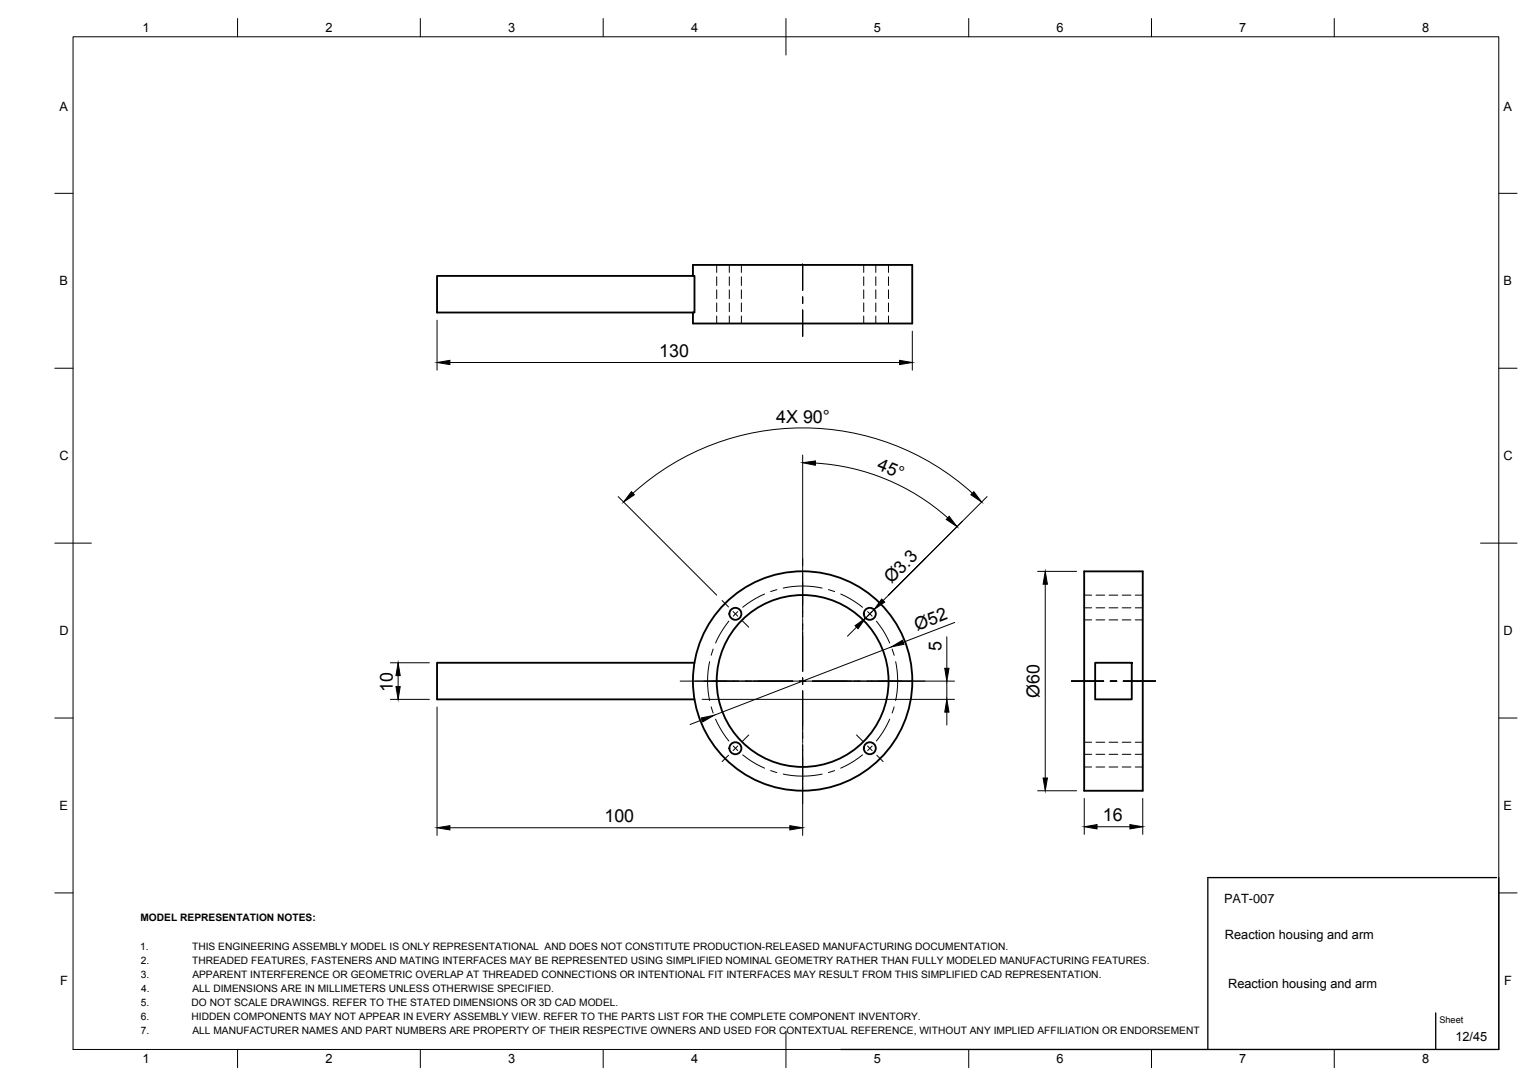
ISO-10303-21;
HEADER;
/* Generated by software containing ST-Developer
 * from STEP Tools, Inc. (www.steptools.com) 
 */

FILE_DESCRIPTION(
/* description */ ('Bearing friction torque test rig'),
/* implementation_level */ '2;1');

FILE_NAME(
/* name */ 'Reaction housing and arm.step',
/* time_stamp */ '2026-10-28T03:24:04-07:00',
/* author */ (''),
/* organization */ (''),
/* preprocessor_version */ 'ST-DEVELOPER v20.2',
/* originating_system */ 'Autodesk Translation Framework v15.17.0.0',
/* authorisation */ '');

FILE_SCHEMA (('AUTOMOTIVE_DESIGN { 1 0 10303 214 3 1 1 }'));
ENDSEC;

DATA;
#10=MECHANICAL_DESIGN_GEOMETRIC_PRESENTATION_REPRESENTATION('',(#546),#14822);
#468=SHAPE_REPRESENTATION_RELATIONSHIP('SRR','None',#15007,#507);
#507=ADVANCED_BREP_SHAPE_REPRESENTATION('',(#600),#14787);
#546=STYLED_ITEM('',(#15263),#600);
#600=MANIFOLD_SOLID_BREP('Body1',#7662);
#744=FACE_BOUND('',#1755,.T.);
#745=FACE_BOUND('',#1757,.T.);
#746=FACE_BOUND('',#1758,.T.);
#747=FACE_BOUND('',#1759,.T.);
#748=FACE_BOUND('',#1760,.T.);
#749=FACE_BOUND('',#1761,.T.);
#750=FACE_BOUND('',#1763,.T.);
#751=FACE_BOUND('',#1764,.T.);
#752=FACE_BOUND('',#1765,.T.);
#753=FACE_BOUND('',#1766,.T.);
#754=FACE_BOUND('',#1767,.T.);
#914=PLANE('',#8392);
#915=PLANE('',#8393);
#916=PLANE('',#8395);
#917=PLANE('',#8397);
#918=PLANE('',#8398);
#919=PLANE('',#8405);
#920=PLANE('',#8406);
#1199=FACE_OUTER_BOUND('',#1744,.T.);
#1200=FACE_OUTER_BOUND('',#1745,.T.);
#1201=FACE_OUTER_BOUND('',#1746,.T.);
#1202=FACE_OUTER_BOUND('',#1747,.T.);
#1203=FACE_OUTER_BOUND('',#1748,.T.);
#1204=FACE_OUTER_BOUND('',#1749,.T.);
#1205=FACE_OUTER_BOUND('',#1750,.T.);
#1206=FACE_OUTER_BOUND('',#1751,.T.);
#1207=FACE_OUTER_BOUND('',#1752,.T.);
#1208=FACE_OUTER_BOUND('',#1753,.T.);
#1209=FACE_OUTER_BOUND('',#1754,.T.);
#1210=FACE_OUTER_BOUND('',#1756,.T.);
#1211=FACE_OUTER_BOUND('',#1762,.T.);
#1744=EDGE_LOOP('',(#5616,#5617,#5618,#5619));
#1745=EDGE_LOOP('',(#5620,#5621,#5622,#5623));
#1746=EDGE_LOOP('',(#5624,#5625,#5626,#5627));
#1747=EDGE_LOOP('',(#5628,#5629,#5630,#5631));
#1748=EDGE_LOOP('',(#5632,#5633,#5634,#5635));
#1749=EDGE_LOOP('',(#5636,#5637,#5638,#5639));
#1750=EDGE_LOOP('',(#5640,#5641,#5642,#5643));
#1751=EDGE_LOOP('',(#5644,#5645,#5646,#5647));
#1752=EDGE_LOOP('',(#5648,#5649,#5650,#5651));
#1753=EDGE_LOOP('',(#5652,#5653,#5654,#5655));
#1754=EDGE_LOOP('',(#5656,#5657,#5658,#5659));
#1755=EDGE_LOOP('',(#5660,#5661,#5662,#5663));
#1756=EDGE_LOOP('',(#5664));
#1757=EDGE_LOOP('',(#5665));
#1758=EDGE_LOOP('',(#5666));
#1759=EDGE_LOOP('',(#5667));
#1760=EDGE_LOOP('',(#5668));
#1761=EDGE_LOOP('',(#5669));
#1762=EDGE_LOOP('',(#5670));
#1763=EDGE_LOOP('',(#5671));
#1764=EDGE_LOOP('',(#5672));
#1765=EDGE_LOOP('',(#5673));
#1766=EDGE_LOOP('',(#5674));
#1767=EDGE_LOOP('',(#5675));
#2325=LINE('',#12162,#2769);
#2326=LINE('',#12168,#2770);
#2327=LINE('',#12174,#2771);
#2328=LINE('',#12180,#2772);
#2329=LINE('',#12185,#2773);
#2330=LINE('',#12187,#2774);
#2331=LINE('',#12189,#2775);
#2332=LINE('',#12190,#2776);
#2333=LINE('',#12195,#2777);
#2334=LINE('',#12196,#2778);
#2335=LINE('',#12201,#2779);
#2336=LINE('',#12202,#2780);
#2337=LINE('',#12204,#2781);
#2338=LINE('',#12205,#2782);
#2339=LINE('',#12211,#2783);
#2340=LINE('',#12217,#2784);
#2769=VECTOR('',#9752,0.165);
#2770=VECTOR('',#9759,0.165);
#2771=VECTOR('',#9766,0.165);
#2772=VECTOR('',#9773,0.165);
#2773=VECTOR('',#9778,1.);
#2774=VECTOR('',#9779,1.);
#2775=VECTOR('',#9780,1.);
#2776=VECTOR('',#9781,1.);
#2777=VECTOR('',#9786,1.);
#2778=VECTOR('',#9787,1.);
#2779=VECTOR('',#9792,1.);
#2780=VECTOR('',#9793,1.);
#2781=VECTOR('',#9796,1.);
#2782=VECTOR('',#9797,1.);
#2783=VECTOR('',#9804,2.35);
#2784=VECTOR('',#9811,3.);
#3229=CIRCLE('',#8381,0.165);
#3230=CIRCLE('',#8382,0.165);
#3231=CIRCLE('',#8384,0.165);
#3232=CIRCLE('',#8385,0.165);
#3233=CIRCLE('',#8387,0.165);
#3234=CIRCLE('',#8388,0.165);
#3235=CIRCLE('',#8390,0.165);
#3236=CIRCLE('',#8391,0.165);
#3237=CIRCLE('',#8394,3.);
#3238=CIRCLE('',#8396,3.);
#3239=CIRCLE('',#8400,2.35);
#3240=CIRCLE('',#8401,2.35);
#3241=CIRCLE('',#8403,3.);
#3242=CIRCLE('',#8404,3.);
#3709=VERTEX_POINT('',#12159);
#3710=VERTEX_POINT('',#12161);
#3711=VERTEX_POINT('',#12165);
#3712=VERTEX_POINT('',#12167);
#3713=VERTEX_POINT('',#12171);
#3714=VERTEX_POINT('',#12173);
#3715=VERTEX_POINT('',#12177);
#3716=VERTEX_POINT('',#12179);
#3717=VERTEX_POINT('',#12183);
#3718=VERTEX_POINT('',#12184);
#3719=VERTEX_POINT('',#12186);
#3720=VERTEX_POINT('',#12188);
#3721=VERTEX_POINT('',#12192);
#3722=VERTEX_POINT('',#12194);
#3723=VERTEX_POINT('',#12198);
#3724=VERTEX_POINT('',#12200);
#3725=VERTEX_POINT('',#12208);
#3726=VERTEX_POINT('',#12210);
#3727=VERTEX_POINT('',#12214);
#3728=VERTEX_POINT('',#12216);
#4434=EDGE_CURVE('',#3709,#3709,#3229,.T.);
#4435=EDGE_CURVE('',#3709,#3710,#2325,.T.);
#4436=EDGE_CURVE('',#3710,#3710,#3230,.T.);
#4437=EDGE_CURVE('',#3711,#3711,#3231,.T.);
#4438=EDGE_CURVE('',#3711,#3712,#2326,.T.);
#4439=EDGE_CURVE('',#3712,#3712,#3232,.T.);
#4440=EDGE_CURVE('',#3713,#3713,#3233,.T.);
#4441=EDGE_CURVE('',#3713,#3714,#2327,.T.);
#4442=EDGE_CURVE('',#3714,#3714,#3234,.T.);
#4443=EDGE_CURVE('',#3715,#3715,#3235,.T.);
#4444=EDGE_CURVE('',#3715,#3716,#2328,.T.);
#4445=EDGE_CURVE('',#3716,#3716,#3236,.T.);
#4446=EDGE_CURVE('',#3717,#3718,#2329,.T.);
#4447=EDGE_CURVE('',#3719,#3717,#2330,.T.);
#4448=EDGE_CURVE('',#3720,#3719,#2331,.T.);
#4449=EDGE_CURVE('',#3718,#3720,#2332,.T.);
#4450=EDGE_CURVE('',#3721,#3717,#3237,.T.);
#4451=EDGE_CURVE('',#3721,#3722,#2333,.T.);
#4452=EDGE_CURVE('',#3722,#3719,#2334,.T.);
#4453=EDGE_CURVE('',#3718,#3723,#3238,.T.);
#4454=EDGE_CURVE('',#3720,#3724,#2335,.T.);
#4455=EDGE_CURVE('',#3724,#3723,#2336,.T.);
#4456=EDGE_CURVE('',#3723,#3721,#2337,.T.);
#4457=EDGE_CURVE('',#3724,#3722,#2338,.T.);
#4458=EDGE_CURVE('',#3725,#3725,#3239,.T.);
#4459=EDGE_CURVE('',#3725,#3726,#2339,.T.);
#4460=EDGE_CURVE('',#3726,#3726,#3240,.T.);
#4461=EDGE_CURVE('',#3727,#3727,#3241,.T.);
#4462=EDGE_CURVE('',#3727,#3728,#2340,.T.);
#4463=EDGE_CURVE('',#3728,#3728,#3242,.T.);
#5616=ORIENTED_EDGE('',*,*,#4434,.F.);
#5617=ORIENTED_EDGE('',*,*,#4435,.T.);
#5618=ORIENTED_EDGE('',*,*,#4436,.F.);
#5619=ORIENTED_EDGE('',*,*,#4435,.F.);
#5620=ORIENTED_EDGE('',*,*,#4437,.F.);
#5621=ORIENTED_EDGE('',*,*,#4438,.T.);
#5622=ORIENTED_EDGE('',*,*,#4439,.F.);
#5623=ORIENTED_EDGE('',*,*,#4438,.F.);
#5624=ORIENTED_EDGE('',*,*,#4440,.F.);
#5625=ORIENTED_EDGE('',*,*,#4441,.T.);
#5626=ORIENTED_EDGE('',*,*,#4442,.F.);
#5627=ORIENTED_EDGE('',*,*,#4441,.F.);
#5628=ORIENTED_EDGE('',*,*,#4443,.F.);
#5629=ORIENTED_EDGE('',*,*,#4444,.T.);
#5630=ORIENTED_EDGE('',*,*,#4445,.F.);
#5631=ORIENTED_EDGE('',*,*,#4444,.F.);
#5632=ORIENTED_EDGE('',*,*,#4446,.F.);
#5633=ORIENTED_EDGE('',*,*,#4447,.F.);
#5634=ORIENTED_EDGE('',*,*,#4448,.F.);
#5635=ORIENTED_EDGE('',*,*,#4449,.F.);
#5636=ORIENTED_EDGE('',*,*,#4450,.F.);
#5637=ORIENTED_EDGE('',*,*,#4451,.T.);
#5638=ORIENTED_EDGE('',*,*,#4452,.T.);
#5639=ORIENTED_EDGE('',*,*,#4447,.T.);
#5640=ORIENTED_EDGE('',*,*,#4453,.F.);
#5641=ORIENTED_EDGE('',*,*,#4449,.T.);
#5642=ORIENTED_EDGE('',*,*,#4454,.T.);
#5643=ORIENTED_EDGE('',*,*,#4455,.T.);
#5644=ORIENTED_EDGE('',*,*,#4456,.F.);
#5645=ORIENTED_EDGE('',*,*,#4455,.F.);
#5646=ORIENTED_EDGE('',*,*,#4457,.T.);
#5647=ORIENTED_EDGE('',*,*,#4451,.F.);
#5648=ORIENTED_EDGE('',*,*,#4454,.F.);
#5649=ORIENTED_EDGE('',*,*,#4448,.T.);
#5650=ORIENTED_EDGE('',*,*,#4452,.F.);
#5651=ORIENTED_EDGE('',*,*,#4457,.F.);
#5652=ORIENTED_EDGE('',*,*,#4458,.F.);
#5653=ORIENTED_EDGE('',*,*,#4459,.T.);
#5654=ORIENTED_EDGE('',*,*,#4460,.T.);
#5655=ORIENTED_EDGE('',*,*,#4459,.F.);
#5656=ORIENTED_EDGE('',*,*,#4461,.F.);
#5657=ORIENTED_EDGE('',*,*,#4462,.T.);
#5658=ORIENTED_EDGE('',*,*,#4463,.T.);
#5659=ORIENTED_EDGE('',*,*,#4462,.F.);
#5660=ORIENTED_EDGE('',*,*,#4456,.T.);
#5661=ORIENTED_EDGE('',*,*,#4450,.T.);
#5662=ORIENTED_EDGE('',*,*,#4446,.T.);
#5663=ORIENTED_EDGE('',*,*,#4453,.T.);
#5664=ORIENTED_EDGE('',*,*,#4461,.T.);
#5665=ORIENTED_EDGE('',*,*,#4458,.T.);
#5666=ORIENTED_EDGE('',*,*,#4445,.T.);
#5667=ORIENTED_EDGE('',*,*,#4442,.T.);
#5668=ORIENTED_EDGE('',*,*,#4439,.T.);
#5669=ORIENTED_EDGE('',*,*,#4436,.T.);
#5670=ORIENTED_EDGE('',*,*,#4463,.F.);
#5671=ORIENTED_EDGE('',*,*,#4460,.F.);
#5672=ORIENTED_EDGE('',*,*,#4443,.T.);
#5673=ORIENTED_EDGE('',*,*,#4440,.T.);
#5674=ORIENTED_EDGE('',*,*,#4437,.T.);
#5675=ORIENTED_EDGE('',*,*,#4434,.T.);
#7104=CYLINDRICAL_SURFACE('',#8380,0.165);
#7105=CYLINDRICAL_SURFACE('',#8383,0.165);
#7106=CYLINDRICAL_SURFACE('',#8386,0.165);
#7107=CYLINDRICAL_SURFACE('',#8389,0.165);
#7108=CYLINDRICAL_SURFACE('',#8399,2.35);
#7109=CYLINDRICAL_SURFACE('',#8402,3.);
#7310=ADVANCED_FACE('',(#1199),#7104,.F.);
#7311=ADVANCED_FACE('',(#1200),#7105,.F.);
#7312=ADVANCED_FACE('',(#1201),#7106,.F.);
#7313=ADVANCED_FACE('',(#1202),#7107,.F.);
#7314=ADVANCED_FACE('',(#1203),#914,.T.);
#7315=ADVANCED_FACE('',(#1204),#915,.T.);
#7316=ADVANCED_FACE('',(#1205),#916,.F.);
#7317=ADVANCED_FACE('',(#1206),#917,.T.);
#7318=ADVANCED_FACE('',(#1207),#918,.T.);
#7319=ADVANCED_FACE('',(#1208),#7108,.F.);
#7320=ADVANCED_FACE('',(#1209,#744),#7109,.T.);
#7321=ADVANCED_FACE('',(#1210,#745,#746,#747,#748,#749),#919,.T.);
#7322=ADVANCED_FACE('',(#1211,#750,#751,#752,#753,#754),#920,.F.);
#7662=CLOSED_SHELL('',(#7310,#7311,#7312,#7313,#7314,#7315,#7316,#7317,
#7318,#7319,#7320,#7321,#7322));
#8379=AXIS2_PLACEMENT_3D('',#12157,#9746,#9747);
#8380=AXIS2_PLACEMENT_3D('',#12158,#9748,#9749);
#8381=AXIS2_PLACEMENT_3D('',#12160,#9750,#9751);
#8382=AXIS2_PLACEMENT_3D('',#12163,#9753,#9754);
#8383=AXIS2_PLACEMENT_3D('',#12164,#9755,#9756);
#8384=AXIS2_PLACEMENT_3D('',#12166,#9757,#9758);
#8385=AXIS2_PLACEMENT_3D('',#12169,#9760,#9761);
#8386=AXIS2_PLACEMENT_3D('',#12170,#9762,#9763);
#8387=AXIS2_PLACEMENT_3D('',#12172,#9764,#9765);
#8388=AXIS2_PLACEMENT_3D('',#12175,#9767,#9768);
#8389=AXIS2_PLACEMENT_3D('',#12176,#9769,#9770);
#8390=AXIS2_PLACEMENT_3D('',#12178,#9771,#9772);
#8391=AXIS2_PLACEMENT_3D('',#12181,#9774,#9775);
#8392=AXIS2_PLACEMENT_3D('',#12182,#9776,#9777);
#8393=AXIS2_PLACEMENT_3D('',#12191,#9782,#9783);
#8394=AXIS2_PLACEMENT_3D('',#12193,#9784,#9785);
#8395=AXIS2_PLACEMENT_3D('',#12197,#9788,#9789);
#8396=AXIS2_PLACEMENT_3D('',#12199,#9790,#9791);
#8397=AXIS2_PLACEMENT_3D('',#12203,#9794,#9795);
#8398=AXIS2_PLACEMENT_3D('',#12206,#9798,#9799);
#8399=AXIS2_PLACEMENT_3D('',#12207,#9800,#9801);
#8400=AXIS2_PLACEMENT_3D('',#12209,#9802,#9803);
#8401=AXIS2_PLACEMENT_3D('',#12212,#9805,#9806);
#8402=AXIS2_PLACEMENT_3D('',#12213,#9807,#9808);
#8403=AXIS2_PLACEMENT_3D('',#12215,#9809,#9810);
#8404=AXIS2_PLACEMENT_3D('',#12218,#9812,#9813);
#8405=AXIS2_PLACEMENT_3D('',#12219,#9814,#9815);
#8406=AXIS2_PLACEMENT_3D('',#12220,#9816,#9817);
#9746=DIRECTION('axis',(0.,0.,1.));
#9747=DIRECTION('refdir',(1.,0.,0.));
#9748=DIRECTION('center_axis',(0.,1.,0.));
#9749=DIRECTION('ref_axis',(1.,0.,0.));
#9750=DIRECTION('center_axis',(0.,1.,0.));
#9751=DIRECTION('ref_axis',(1.,0.,0.));
#9752=DIRECTION('',(0.,1.,0.));
#9753=DIRECTION('center_axis',(0.,-1.,0.));
#9754=DIRECTION('ref_axis',(1.,0.,0.));
#9755=DIRECTION('center_axis',(0.,1.,0.));
#9756=DIRECTION('ref_axis',(1.,0.,0.));
#9757=DIRECTION('center_axis',(0.,1.,0.));
#9758=DIRECTION('ref_axis',(1.,0.,0.));
#9759=DIRECTION('',(0.,1.,0.));
#9760=DIRECTION('center_axis',(0.,-1.,0.));
#9761=DIRECTION('ref_axis',(1.,0.,0.));
#9762=DIRECTION('center_axis',(0.,1.,0.));
#9763=DIRECTION('ref_axis',(1.,0.,0.));
#9764=DIRECTION('center_axis',(0.,1.,0.));
#9765=DIRECTION('ref_axis',(1.,0.,0.));
#9766=DIRECTION('',(0.,1.,0.));
#9767=DIRECTION('center_axis',(0.,-1.,0.));
#9768=DIRECTION('ref_axis',(1.,0.,0.));
#9769=DIRECTION('center_axis',(0.,1.,0.));
#9770=DIRECTION('ref_axis',(1.,0.,0.));
#9771=DIRECTION('center_axis',(0.,1.,0.));
#9772=DIRECTION('ref_axis',(1.,0.,0.));
#9773=DIRECTION('',(0.,1.,0.));
#9774=DIRECTION('center_axis',(0.,-1.,0.));
#9775=DIRECTION('ref_axis',(1.,0.,0.));
#9776=DIRECTION('center_axis',(0.,0.,-1.));
#9777=DIRECTION('ref_axis',(-1.,0.,0.));
#9778=DIRECTION('',(0.,-1.,0.));
#9779=DIRECTION('',(-1.,0.,0.));
#9780=DIRECTION('',(0.,1.,0.));
#9781=DIRECTION('',(1.,0.,0.));
#9782=DIRECTION('center_axis',(0.,1.,0.));
#9783=DIRECTION('ref_axis',(0.,0.,1.));
#9784=DIRECTION('center_axis',(0.,1.,0.));
#9785=DIRECTION('ref_axis',(1.,0.,0.));
#9786=DIRECTION('',(1.,0.,0.));
#9787=DIRECTION('',(0.,0.,-1.));
#9788=DIRECTION('center_axis',(0.,1.,0.));
#9789=DIRECTION('ref_axis',(1.,0.,0.));
#9790=DIRECTION('center_axis',(0.,-1.,0.));
#9791=DIRECTION('ref_axis',(1.,0.,0.));
#9792=DIRECTION('',(0.,0.,1.));
#9793=DIRECTION('',(-1.,0.,0.));
#9794=DIRECTION('center_axis',(0.,0.,1.));
#9795=DIRECTION('ref_axis',(1.,0.,0.));
#9796=DIRECTION('',(0.,1.,0.));
#9797=DIRECTION('',(0.,1.,0.));
#9798=DIRECTION('center_axis',(1.,0.,0.));
#9799=DIRECTION('ref_axis',(0.,0.,-1.));
#9800=DIRECTION('center_axis',(0.,1.,0.));
#9801=DIRECTION('ref_axis',(1.,0.,0.));
#9802=DIRECTION('center_axis',(0.,-1.,0.));
#9803=DIRECTION('ref_axis',(1.,0.,0.));
#9804=DIRECTION('',(0.,-1.,0.));
#9805=DIRECTION('center_axis',(0.,-1.,0.));
#9806=DIRECTION('ref_axis',(1.,0.,0.));
#9807=DIRECTION('center_axis',(0.,1.,0.));
#9808=DIRECTION('ref_axis',(1.,0.,0.));
#9809=DIRECTION('center_axis',(0.,1.,0.));
#9810=DIRECTION('ref_axis',(1.,0.,0.));
#9811=DIRECTION('',(0.,-1.,0.));
#9812=DIRECTION('center_axis',(0.,1.,0.));
#9813=DIRECTION('ref_axis',(1.,0.,0.));
#9814=DIRECTION('center_axis',(0.,1.,0.));
#9815=DIRECTION('ref_axis',(1.,0.,0.));
#9816=DIRECTION('center_axis',(0.,1.,0.));
#9817=DIRECTION('ref_axis',(1.,0.,0.));
#12157=CARTESIAN_POINT('',(0.,0.,0.));
#12158=CARTESIAN_POINT('Origin',(-1.83847763108502,-0.9,5.16152236891498));
#12159=CARTESIAN_POINT('',(-2.00347763108502,-0.8,5.16152236891498));
#12160=CARTESIAN_POINT('Origin',(-1.83847763108502,-0.8,5.16152236891498));
#12161=CARTESIAN_POINT('',(-2.00347763108502,0.8,5.16152236891498));
#12162=CARTESIAN_POINT('',(-2.00347763108502,-0.9,5.16152236891498));
#12163=CARTESIAN_POINT('Origin',(-1.83847763108502,0.8,5.16152236891498));
#12164=CARTESIAN_POINT('Origin',(-1.83847763108502,-0.9,8.83847763108502));
#12165=CARTESIAN_POINT('',(-2.00347763108502,-0.8,8.83847763108502));
#12166=CARTESIAN_POINT('Origin',(-1.83847763108502,-0.8,8.83847763108502));
#12167=CARTESIAN_POINT('',(-2.00347763108502,0.8,8.83847763108502));
#12168=CARTESIAN_POINT('',(-2.00347763108502,-0.9,8.83847763108502));
#12169=CARTESIAN_POINT('Origin',(-1.83847763108502,0.8,8.83847763108502));
#12170=CARTESIAN_POINT('Origin',(1.83847763108502,-0.9,8.83847763108502));
#12171=CARTESIAN_POINT('',(1.67347763108502,-0.8,8.83847763108502));
#12172=CARTESIAN_POINT('Origin',(1.83847763108502,-0.8,8.83847763108502));
#12173=CARTESIAN_POINT('',(1.67347763108502,0.8,8.83847763108502));
#12174=CARTESIAN_POINT('',(1.67347763108502,-0.9,8.83847763108502));
#12175=CARTESIAN_POINT('Origin',(1.83847763108502,0.8,8.83847763108502));
#12176=CARTESIAN_POINT('Origin',(1.83847763108502,-0.9,5.16152236891498));
#12177=CARTESIAN_POINT('',(1.67347763108502,-0.8,5.16152236891498));
#12178=CARTESIAN_POINT('Origin',(1.83847763108502,-0.8,5.16152236891498));
#12179=CARTESIAN_POINT('',(1.67347763108502,0.8,5.16152236891498));
#12180=CARTESIAN_POINT('',(1.67347763108502,-0.9,5.16152236891498));
#12181=CARTESIAN_POINT('Origin',(1.83847763108502,0.8,5.16152236891498));
#12182=CARTESIAN_POINT('Origin',(10.,-0.5,6.5));
#12183=CARTESIAN_POINT('',(2.95803989154981,0.5,6.5));
#12184=CARTESIAN_POINT('',(2.95803989154981,-0.5,6.5));
#12185=CARTESIAN_POINT('',(2.95803989154981,-0.8,6.5));
#12186=CARTESIAN_POINT('',(10.,0.5,6.5));
#12187=CARTESIAN_POINT('',(2.,0.5,6.5));
#12188=CARTESIAN_POINT('',(10.,-0.5,6.5));
#12189=CARTESIAN_POINT('',(10.,-0.5,6.5));
#12190=CARTESIAN_POINT('',(2.,-0.5,6.5));
#12191=CARTESIAN_POINT('Origin',(6.,0.5,7.));
#12192=CARTESIAN_POINT('',(2.95803989154981,0.5,7.5));
#12193=CARTESIAN_POINT('Origin',(0.,0.5,7.));
#12194=CARTESIAN_POINT('',(10.,0.5,7.5));
#12195=CARTESIAN_POINT('',(10.,0.5,7.5));
#12196=CARTESIAN_POINT('',(10.,0.5,6.5));
#12197=CARTESIAN_POINT('Origin',(6.,-0.5,7.));
#12198=CARTESIAN_POINT('',(2.95803989154981,-0.5,7.5));
#12199=CARTESIAN_POINT('Origin',(0.,-0.5,7.));
#12200=CARTESIAN_POINT('',(10.,-0.5,7.5));
#12201=CARTESIAN_POINT('',(10.,-0.5,6.5));
#12202=CARTESIAN_POINT('',(10.,-0.5,7.5));
#12203=CARTESIAN_POINT('Origin',(2.,-0.5,7.5));
#12204=CARTESIAN_POINT('',(2.95803989154981,-0.8,7.5));
#12205=CARTESIAN_POINT('',(10.,-0.5,7.5));
#12206=CARTESIAN_POINT('Origin',(10.,-0.5,7.5));
#12207=CARTESIAN_POINT('Origin',(0.,-0.8,7.));
#12208=CARTESIAN_POINT('',(-2.35,0.8,7.));
#12209=CARTESIAN_POINT('Origin',(0.,0.8,7.));
#12210=CARTESIAN_POINT('',(-2.35,-0.8,7.));
#12211=CARTESIAN_POINT('',(-2.35,-0.8,7.));
#12212=CARTESIAN_POINT('Origin',(0.,-0.8,7.));
#12213=CARTESIAN_POINT('Origin',(0.,-0.8,7.));
#12214=CARTESIAN_POINT('',(-3.,0.8,7.));
#12215=CARTESIAN_POINT('Origin',(0.,0.8,7.));
#12216=CARTESIAN_POINT('',(-3.,-0.8,7.));
#12217=CARTESIAN_POINT('',(-3.,-0.8,7.));
#12218=CARTESIAN_POINT('Origin',(0.,-0.8,7.));
#12219=CARTESIAN_POINT('Origin',(0.,0.8,7.));
#12220=CARTESIAN_POINT('Origin',(0.,-0.8,7.));
#14742=UNCERTAINTY_MEASURE_WITH_UNIT(LENGTH_MEASURE(0.001),#14823,
'DISTANCE_ACCURACY_VALUE',
'Maximum model space distance between geometric entities at asserted c
onnectivities');
#14777=UNCERTAINTY_MEASURE_WITH_UNIT(LENGTH_MEASURE(0.001),#14823,
'DISTANCE_ACCURACY_VALUE',
'Maximum model space distance between geometric entities at asserted c
onnectivities');
#14787=(
GEOMETRIC_REPRESENTATION_CONTEXT(3)
GLOBAL_UNCERTAINTY_ASSIGNED_CONTEXT((#14742))
GLOBAL_UNIT_ASSIGNED_CONTEXT((#14823,#14825,#14826))
REPRESENTATION_CONTEXT('','3D')
);
#14822=(
GEOMETRIC_REPRESENTATION_CONTEXT(3)
GLOBAL_UNCERTAINTY_ASSIGNED_CONTEXT((#14777))
GLOBAL_UNIT_ASSIGNED_CONTEXT((#14823,#14825,#14826))
REPRESENTATION_CONTEXT('','3D')
);
#14823=(
LENGTH_UNIT()
NAMED_UNIT(*)
SI_UNIT(.CENTI.,.METRE.)
);
#14825=(
NAMED_UNIT(*)
PLANE_ANGLE_UNIT()
SI_UNIT($,.RADIAN.)
);
#14826=(
NAMED_UNIT(*)
SI_UNIT($,.STERADIAN.)
SOLID_ANGLE_UNIT()
);
#14836=SHAPE_DEFINITION_REPRESENTATION(#14880,#15007);
#14880=PRODUCT_DEFINITION_SHAPE('',$,#15052);
#15007=SHAPE_REPRESENTATION('',(#8379),#14787);
#15042=PRODUCT_DEFINITION_CONTEXT('part definition',#15176,'design');
#15052=PRODUCT_DEFINITION('Reaction housing and arm',
'Reaction housing and arm',#15096,#15042);
#15096=PRODUCT_DEFINITION_FORMATION('',$,#15187);
#15176=APPLICATION_CONTEXT(
'Core Data for Automotive Mechanical Design Process');
#15177=PRODUCT_CONTEXT('part definition',#15176,'mechanical');
#15187=PRODUCT('Reaction housing and arm','Reaction housing and arm',
'Reaction housing and arm',(#15177));
#15257=COLOUR_RGB('Dark Blue',0.08,0.2,0.34);
#15258=FILL_AREA_STYLE_COLOUR('',#15257);
#15259=FILL_AREA_STYLE('',(#15258));
#15260=SURFACE_STYLE_FILL_AREA(#15259);
#15261=SURFACE_SIDE_STYLE('',(#15260));
#15262=SURFACE_STYLE_USAGE(.BOTH.,#15261);
#15263=PRESENTATION_STYLE_ASSIGNMENT((#15262));
ENDSEC;
END-ISO-10303-21;
